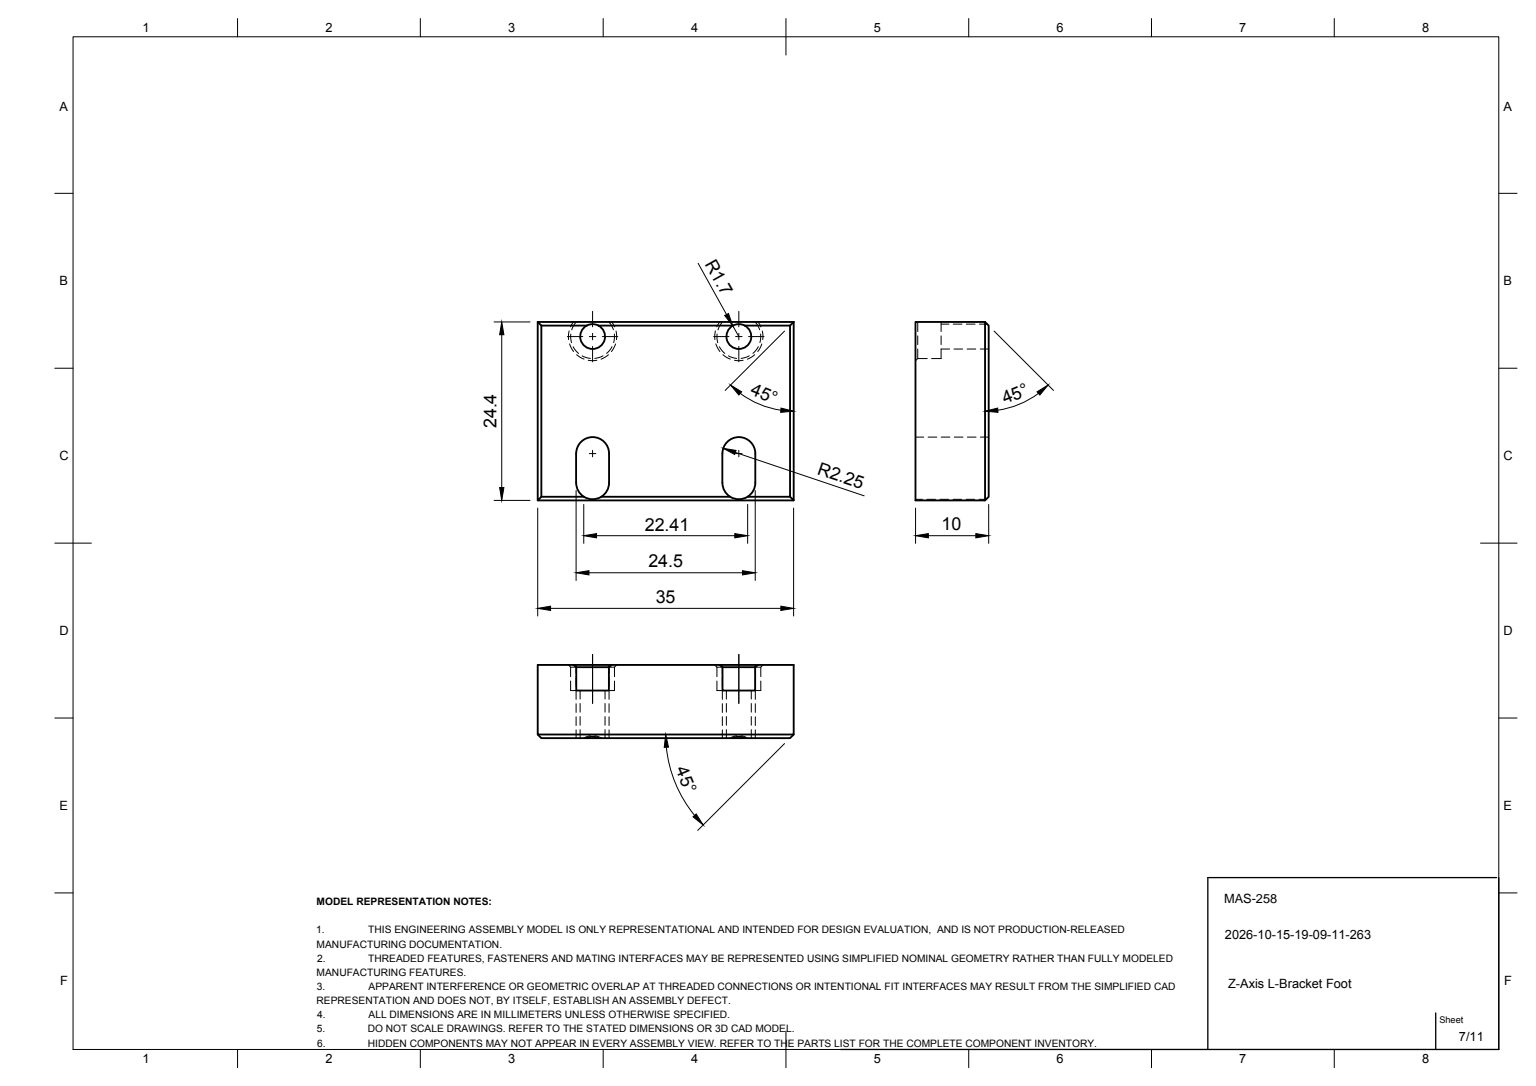
ISO-10303-21;
HEADER;
/* Generated by software containing ST-Developer
 * from STEP Tools, Inc. (www.steptools.com) 
 */

FILE_DESCRIPTION(
/* description */ (''),
/* implementation_level */ '2;1');

FILE_NAME(
/* name */ 'Z-Axis L-Bracket Foot.step',
/* time_stamp */ '2026-10-15T12:29:06-07:00',
/* author */ (''),
/* organization */ (''),
/* preprocessor_version */ 'ST-DEVELOPER v20.2',
/* originating_system */ 'Autodesk Translation Framework v15.15.0.0',
/* authorisation */ '');

FILE_SCHEMA (('AUTOMOTIVE_DESIGN { 1 0 10303 214 3 1 1 }'));
ENDSEC;

DATA;
#10=MECHANICAL_DESIGN_GEOMETRIC_PRESENTATION_REPRESENTATION('',(#1746),#135282);
#100=(
BOUNDED_CURVE()
B_SPLINE_CURVE(2,(#76990,#76991,#76992),.UNSPECIFIED.,.F.,.F.)
B_SPLINE_CURVE_WITH_KNOTS((3,3),(0.557415897727321,0.585832740635072),
 .UNSPECIFIED.)
CURVE()
GEOMETRIC_REPRESENTATION_ITEM()
RATIONAL_B_SPLINE_CURVE((1.06,1.03152938818342,1.))
REPRESENTATION_ITEM('')
);
#101=(
BOUNDED_CURVE()
B_SPLINE_CURVE(2,(#76996,#76997,#76998),.UNSPECIFIED.,.F.,.F.)
B_SPLINE_CURVE_WITH_KNOTS((3,3),(0.,0.0284168429077509),.UNSPECIFIED.)
CURVE()
GEOMETRIC_REPRESENTATION_ITEM()
RATIONAL_B_SPLINE_CURVE((1.,1.03152938818342,1.06))
REPRESENTATION_ITEM('')
);
#102=(
BOUNDED_CURVE()
B_SPLINE_CURVE(2,(#77032,#77033,#77034),.UNSPECIFIED.,.F.,.F.)
B_SPLINE_CURVE_WITH_KNOTS((3,3),(0.557415897727321,0.585832740635072),
 .UNSPECIFIED.)
CURVE()
GEOMETRIC_REPRESENTATION_ITEM()
RATIONAL_B_SPLINE_CURVE((1.06,1.03152938818342,1.))
REPRESENTATION_ITEM('')
);
#103=(
BOUNDED_CURVE()
B_SPLINE_CURVE(2,(#77036,#77037,#77038),.UNSPECIFIED.,.F.,.F.)
B_SPLINE_CURVE_WITH_KNOTS((3,3),(0.,0.028416842907751),.UNSPECIFIED.)
CURVE()
GEOMETRIC_REPRESENTATION_ITEM()
RATIONAL_B_SPLINE_CURVE((1.,1.03152938818342,1.06))
REPRESENTATION_ITEM('')
);
#300=ELLIPSE('',#33382,2.40416305603426,1.7);
#301=ELLIPSE('',#33386,2.40416305603426,1.7);
#302=ELLIPSE('',#33391,3.18198051533946,2.25);
#303=ELLIPSE('',#33399,3.18198051533947,2.25);
#1720=SHAPE_REPRESENTATION_RELATIONSHIP('SRR','None',#135344,#1733);
#1733=ADVANCED_BREP_SHAPE_REPRESENTATION('',(#1759),#135276);
#1746=STYLED_ITEM('',(#135418),#1759);
#1759=MANIFOLD_SOLID_BREP('Body1',#32082);
#1848=CYLINDRICAL_SURFACE('',#33372,3.);
#1849=CYLINDRICAL_SURFACE('',#33376,3.);
#1850=CYLINDRICAL_SURFACE('',#33380,1.7);
#1851=CYLINDRICAL_SURFACE('',#33384,1.7);
#1852=CYLINDRICAL_SURFACE('',#33390,2.25);
#1853=CYLINDRICAL_SURFACE('',#33395,2.25);
#1854=CYLINDRICAL_SURFACE('',#33398,2.25);
#1855=CYLINDRICAL_SURFACE('',#33403,2.25);
#2210=FACE_BOUND('',#6520,.T.);
#2211=FACE_BOUND('',#6521,.T.);
#2212=FACE_BOUND('',#6526,.T.);
#2213=FACE_BOUND('',#6529,.T.);
#3026=PLANE('',#33363);
#3027=PLANE('',#33371);
#3028=PLANE('',#33374);
#3029=PLANE('',#33378);
#3030=PLANE('',#33388);
#3031=PLANE('',#33389);
#3032=PLANE('',#33394);
#3033=PLANE('',#33397);
#3034=PLANE('',#33402);
#3035=PLANE('',#33405);
#3036=PLANE('',#33406);
#3037=PLANE('',#33407);
#3038=PLANE('',#33408);
#3039=PLANE('',#33409);
#3040=PLANE('',#33410);
#3041=PLANE('',#33411);
#4570=FACE_OUTER_BOUND('',#6518,.T.);
#4571=FACE_OUTER_BOUND('',#6519,.T.);
#4572=FACE_OUTER_BOUND('',#6522,.T.);
#4573=FACE_OUTER_BOUND('',#6523,.T.);
#4574=FACE_OUTER_BOUND('',#6524,.T.);
#4575=FACE_OUTER_BOUND('',#6525,.T.);
#4576=FACE_OUTER_BOUND('',#6527,.T.);
#4577=FACE_OUTER_BOUND('',#6528,.T.);
#4578=FACE_OUTER_BOUND('',#6530,.T.);
#4579=FACE_OUTER_BOUND('',#6531,.T.);
#4580=FACE_OUTER_BOUND('',#6532,.T.);
#4581=FACE_OUTER_BOUND('',#6533,.T.);
#4582=FACE_OUTER_BOUND('',#6534,.T.);
#4583=FACE_OUTER_BOUND('',#6535,.T.);
#4584=FACE_OUTER_BOUND('',#6536,.T.);
#4585=FACE_OUTER_BOUND('',#6537,.T.);
#4586=FACE_OUTER_BOUND('',#6538,.T.);
#4587=FACE_OUTER_BOUND('',#6539,.T.);
#4588=FACE_OUTER_BOUND('',#6540,.T.);
#4589=FACE_OUTER_BOUND('',#6541,.T.);
#4590=FACE_OUTER_BOUND('',#6542,.T.);
#4591=FACE_OUTER_BOUND('',#6543,.T.);
#4592=FACE_OUTER_BOUND('',#6544,.T.);
#4593=FACE_OUTER_BOUND('',#6545,.T.);
#4594=FACE_OUTER_BOUND('',#6546,.T.);
#4595=FACE_OUTER_BOUND('',#6547,.T.);
#6518=EDGE_LOOP('',(#27186,#27187,#27188,#27189));
#6519=EDGE_LOOP('',(#27190,#27191,#27192,#27193,#27194,#27195,#27196,#27197));
#6520=EDGE_LOOP('',(#27198,#27199,#27200,#27201));
#6521=EDGE_LOOP('',(#27202,#27203,#27204,#27205));
#6522=EDGE_LOOP('',(#27206,#27207,#27208,#27209));
#6523=EDGE_LOOP('',(#27210,#27211,#27212,#27213,#27214,#27215,#27216,#27217,
#27218,#27219,#27220,#27221,#27222,#27223,#27224,#27225));
#6524=EDGE_LOOP('',(#27226,#27227,#27228,#27229));
#6525=EDGE_LOOP('',(#27230,#27231));
#6526=EDGE_LOOP('',(#27232));
#6527=EDGE_LOOP('',(#27233,#27234,#27235,#27236));
#6528=EDGE_LOOP('',(#27237,#27238));
#6529=EDGE_LOOP('',(#27239));
#6530=EDGE_LOOP('',(#27240,#27241,#27242,#27243,#27244,#27245));
#6531=EDGE_LOOP('',(#27246,#27247,#27248,#27249,#27250,#27251));
#6532=EDGE_LOOP('',(#27252,#27253,#27254,#27255,#27256,#27257,#27258,#27259));
#6533=EDGE_LOOP('',(#27260,#27261,#27262,#27263));
#6534=EDGE_LOOP('',(#27264,#27265,#27266,#27267,#27268,#27269));
#6535=EDGE_LOOP('',(#27270,#27271,#27272,#27273));
#6536=EDGE_LOOP('',(#27274,#27275,#27276,#27277));
#6537=EDGE_LOOP('',(#27278,#27279,#27280,#27281));
#6538=EDGE_LOOP('',(#27282,#27283,#27284,#27285,#27286,#27287));
#6539=EDGE_LOOP('',(#27288,#27289,#27290,#27291));
#6540=EDGE_LOOP('',(#27292,#27293,#27294,#27295));
#6541=EDGE_LOOP('',(#27296,#27297,#27298,#27299,#27300,#27301,#27302,#27303,
#27304,#27305,#27306,#27307,#27308,#27309,#27310,#27311,#27312,#27313,#27314,
#27315,#27316,#27317));
#6542=EDGE_LOOP('',(#27318,#27319,#27320,#27321));
#6543=EDGE_LOOP('',(#27322,#27323,#27324,#27325));
#6544=EDGE_LOOP('',(#27326,#27327,#27328,#27329,#27330,#27331,#27332,#27333));
#6545=EDGE_LOOP('',(#27334,#27335,#27336,#27337));
#6546=EDGE_LOOP('',(#27338,#27339,#27340,#27341));
#6547=EDGE_LOOP('',(#27342,#27343,#27344,#27345));
#9216=LINE('',#77002,#12053);
#9217=LINE('',#77006,#12054);
#9218=LINE('',#77008,#12055);
#9219=LINE('',#77010,#12056);
#9220=LINE('',#77012,#12057);
#9221=LINE('',#77013,#12058);
#9222=LINE('',#77016,#12059);
#9223=LINE('',#77020,#12060);
#9224=LINE('',#77024,#12061);
#9225=LINE('',#77028,#12062);
#9226=LINE('',#77042,#12063);
#9227=LINE('',#77044,#12064);
#9228=LINE('',#77045,#12065);
#9229=LINE('',#77047,#12066);
#9230=LINE('',#77049,#12067);
#9231=LINE('',#77050,#12068);
#9232=LINE('',#77052,#12069);
#9233=LINE('',#77054,#12070);
#9234=LINE('',#77055,#12071);
#9235=LINE('',#77068,#12072);
#9236=LINE('',#77076,#12073);
#9237=LINE('',#77084,#12074);
#9238=LINE('',#77085,#12075);
#9239=LINE('',#77087,#12076);
#9240=LINE('',#77088,#12077);
#9241=LINE('',#77089,#12078);
#9242=LINE('',#77093,#12079);
#9243=LINE('',#77094,#12080);
#9244=LINE('',#77095,#12081);
#9245=LINE('',#77102,#12082);
#9246=LINE('',#77106,#12083);
#9247=LINE('',#77107,#12084);
#9248=LINE('',#77113,#12085);
#9249=LINE('',#77114,#12086);
#9250=LINE('',#77115,#12087);
#9251=LINE('',#77122,#12088);
#9252=LINE('',#77126,#12089);
#9253=LINE('',#77127,#12090);
#9254=LINE('',#77132,#12091);
#9255=LINE('',#77133,#12092);
#9256=LINE('',#77134,#12093);
#9257=LINE('',#77136,#12094);
#9258=LINE('',#77137,#12095);
#9259=LINE('',#77140,#12096);
#9260=LINE('',#77141,#12097);
#9261=LINE('',#77144,#12098);
#9262=LINE('',#77145,#12099);
#9263=LINE('',#77147,#12100);
#9264=LINE('',#77149,#12101);
#9265=LINE('',#77150,#12102);
#12053=VECTOR('',#38634,10.);
#12054=VECTOR('',#38637,10.);
#12055=VECTOR('',#38638,10.);
#12056=VECTOR('',#38639,10.);
#12057=VECTOR('',#38640,10.);
#12058=VECTOR('',#38641,10.);
#12059=VECTOR('',#38642,10.);
#12060=VECTOR('',#38645,10.);
#12061=VECTOR('',#38648,10.);
#12062=VECTOR('',#38651,10.);
#12063=VECTOR('',#38660,10.);
#12064=VECTOR('',#38661,10.);
#12065=VECTOR('',#38662,10.);
#12066=VECTOR('',#38663,10.);
#12067=VECTOR('',#38664,10.);
#12068=VECTOR('',#38665,10.);
#12069=VECTOR('',#38666,10.);
#12070=VECTOR('',#38667,10.);
#12071=VECTOR('',#38668,10.);
#12072=VECTOR('',#38687,1.7);
#12073=VECTOR('',#38696,1.7);
#12074=VECTOR('',#38705,10.);
#12075=VECTOR('',#38706,10.);
#12076=VECTOR('',#38707,10.);
#12077=VECTOR('',#38708,10.);
#12078=VECTOR('',#38709,10.);
#12079=VECTOR('',#38712,10.);
#12080=VECTOR('',#38713,10.);
#12081=VECTOR('',#38714,10.);
#12082=VECTOR('',#38721,10.);
#12083=VECTOR('',#38726,10.);
#12084=VECTOR('',#38727,10.);
#12085=VECTOR('',#38734,10.);
#12086=VECTOR('',#38735,10.);
#12087=VECTOR('',#38736,10.);
#12088=VECTOR('',#38743,10.);
#12089=VECTOR('',#38748,10.);
#12090=VECTOR('',#38749,10.);
#12091=VECTOR('',#38756,10.);
#12092=VECTOR('',#38757,10.);
#12093=VECTOR('',#38758,10.);
#12094=VECTOR('',#38759,10.);
#12095=VECTOR('',#38760,10.);
#12096=VECTOR('',#38763,10.);
#12097=VECTOR('',#38764,10.);
#12098=VECTOR('',#38767,10.);
#12099=VECTOR('',#38768,10.);
#12100=VECTOR('',#38771,10.);
#12101=VECTOR('',#38774,10.);
#12102=VECTOR('',#38775,10.);
#12932=CIRCLE('',#33361,3.3);
#12933=CIRCLE('',#33362,3.);
#12934=CIRCLE('',#33364,3.3);
#12935=CIRCLE('',#33365,2.25);
#12936=CIRCLE('',#33366,2.25);
#12937=CIRCLE('',#33367,2.25);
#12938=CIRCLE('',#33368,2.25);
#12939=CIRCLE('',#33370,3.);
#12940=CIRCLE('',#33373,3.);
#12941=CIRCLE('',#33375,1.7);
#12942=CIRCLE('',#33377,3.);
#12943=CIRCLE('',#33379,1.7);
#12944=CIRCLE('',#33381,1.7);
#12945=CIRCLE('',#33383,1.7);
#12946=CIRCLE('',#33385,1.7);
#12947=CIRCLE('',#33387,1.7);
#12948=CIRCLE('',#33392,2.25);
#12949=CIRCLE('',#33393,2.25);
#12950=CIRCLE('',#33396,2.25);
#12951=CIRCLE('',#33400,2.25);
#12952=CIRCLE('',#33401,2.25);
#12953=CIRCLE('',#33404,2.25);
#15317=VERTEX_POINT('',#76988);
#15318=VERTEX_POINT('',#76989);
#15319=VERTEX_POINT('',#76993);
#15320=VERTEX_POINT('',#76995);
#15321=VERTEX_POINT('',#77001);
#15322=VERTEX_POINT('',#77003);
#15323=VERTEX_POINT('',#77005);
#15324=VERTEX_POINT('',#77007);
#15325=VERTEX_POINT('',#77009);
#15326=VERTEX_POINT('',#77011);
#15327=VERTEX_POINT('',#77014);
#15328=VERTEX_POINT('',#77015);
#15329=VERTEX_POINT('',#77017);
#15330=VERTEX_POINT('',#77019);
#15331=VERTEX_POINT('',#77022);
#15332=VERTEX_POINT('',#77023);
#15333=VERTEX_POINT('',#77025);
#15334=VERTEX_POINT('',#77027);
#15335=VERTEX_POINT('',#77031);
#15336=VERTEX_POINT('',#77035);
#15337=VERTEX_POINT('',#77041);
#15338=VERTEX_POINT('',#77043);
#15339=VERTEX_POINT('',#77046);
#15340=VERTEX_POINT('',#77048);
#15341=VERTEX_POINT('',#77051);
#15342=VERTEX_POINT('',#77053);
#15343=VERTEX_POINT('',#77059);
#15344=VERTEX_POINT('',#77064);
#15345=VERTEX_POINT('',#77067);
#15346=VERTEX_POINT('',#77069);
#15347=VERTEX_POINT('',#77071);
#15348=VERTEX_POINT('',#77075);
#15349=VERTEX_POINT('',#77077);
#15350=VERTEX_POINT('',#77079);
#15351=VERTEX_POINT('',#77083);
#15352=VERTEX_POINT('',#77086);
#15353=VERTEX_POINT('',#77091);
#15354=VERTEX_POINT('',#77092);
#15355=VERTEX_POINT('',#77097);
#15356=VERTEX_POINT('',#77098);
#15357=VERTEX_POINT('',#77100);
#15358=VERTEX_POINT('',#77105);
#15359=VERTEX_POINT('',#77111);
#15360=VERTEX_POINT('',#77112);
#15361=VERTEX_POINT('',#77117);
#15362=VERTEX_POINT('',#77118);
#15363=VERTEX_POINT('',#77120);
#15364=VERTEX_POINT('',#77125);
#15365=VERTEX_POINT('',#77131);
#15366=VERTEX_POINT('',#77135);
#15367=VERTEX_POINT('',#77139);
#15368=VERTEX_POINT('',#77143);
#19444=EDGE_CURVE('',#15317,#15318,#100,.T.);
#19445=EDGE_CURVE('',#15318,#15319,#12932,.T.);
#19446=EDGE_CURVE('',#15319,#15320,#101,.T.);
#19447=EDGE_CURVE('',#15320,#15317,#12933,.T.);
#19448=EDGE_CURVE('',#15318,#15321,#9216,.T.);
#19449=EDGE_CURVE('',#15322,#15321,#12934,.T.);
#19450=EDGE_CURVE('',#15322,#15323,#9217,.T.);
#19451=EDGE_CURVE('',#15323,#15324,#9218,.T.);
#19452=EDGE_CURVE('',#15324,#15325,#9219,.T.);
#19453=EDGE_CURVE('',#15325,#15326,#9220,.T.);
#19454=EDGE_CURVE('',#15326,#15319,#9221,.T.);
#19455=EDGE_CURVE('',#15327,#15328,#9222,.T.);
#19456=EDGE_CURVE('',#15328,#15329,#12935,.T.);
#19457=EDGE_CURVE('',#15329,#15330,#9223,.T.);
#19458=EDGE_CURVE('',#15330,#15327,#12936,.T.);
#19459=EDGE_CURVE('',#15331,#15332,#9224,.T.);
#19460=EDGE_CURVE('',#15332,#15333,#12937,.T.);
#19461=EDGE_CURVE('',#15333,#15334,#9225,.T.);
#19462=EDGE_CURVE('',#15334,#15331,#12938,.T.);
#19463=EDGE_CURVE('',#15335,#15322,#102,.T.);
#19464=EDGE_CURVE('',#15321,#15336,#103,.T.);
#19465=EDGE_CURVE('',#15336,#15335,#12939,.T.);
#19466=EDGE_CURVE('',#15326,#15337,#9226,.T.);
#19467=EDGE_CURVE('',#15338,#15337,#9227,.T.);
#19468=EDGE_CURVE('',#15323,#15338,#9228,.T.);
#19469=EDGE_CURVE('',#15335,#15339,#9229,.T.);
#19470=EDGE_CURVE('',#15339,#15340,#9230,.T.);
#19471=EDGE_CURVE('',#15340,#15336,#9231,.T.);
#19472=EDGE_CURVE('',#15317,#15341,#9232,.T.);
#19473=EDGE_CURVE('',#15341,#15342,#9233,.T.);
#19474=EDGE_CURVE('',#15342,#15320,#9234,.T.);
#19475=EDGE_CURVE('',#15340,#15339,#12940,.T.);
#19476=EDGE_CURVE('',#15343,#15343,#12941,.T.);
#19477=EDGE_CURVE('',#15342,#15341,#12942,.T.);
#19478=EDGE_CURVE('',#15344,#15344,#12943,.T.);
#19479=EDGE_CURVE('',#15343,#15345,#9235,.T.);
#19480=EDGE_CURVE('',#15346,#15345,#12944,.T.);
#19481=EDGE_CURVE('',#15347,#15346,#300,.T.);
#19482=EDGE_CURVE('',#15345,#15347,#12945,.T.);
#19483=EDGE_CURVE('',#15344,#15348,#9236,.T.);
#19484=EDGE_CURVE('',#15349,#15348,#12946,.T.);
#19485=EDGE_CURVE('',#15350,#15349,#301,.T.);
#19486=EDGE_CURVE('',#15348,#15350,#12947,.T.);
#19487=EDGE_CURVE('',#15346,#15351,#9237,.T.);
#19488=EDGE_CURVE('',#15351,#15338,#9238,.T.);
#19489=EDGE_CURVE('',#15352,#15337,#9239,.T.);
#19490=EDGE_CURVE('',#15352,#15350,#9240,.T.);
#19491=EDGE_CURVE('',#15349,#15347,#9241,.T.);
#19492=EDGE_CURVE('',#15353,#15354,#9242,.T.);
#19493=EDGE_CURVE('',#15353,#15332,#9243,.T.);
#19494=EDGE_CURVE('',#15354,#15331,#9244,.T.);
#19495=EDGE_CURVE('',#15355,#15356,#302,.T.);
#19496=EDGE_CURVE('',#15357,#15355,#12948,.T.);
#19497=EDGE_CURVE('',#15357,#15333,#9245,.T.);
#19498=EDGE_CURVE('',#15356,#15353,#12949,.T.);
#19499=EDGE_CURVE('',#15358,#15357,#9246,.T.);
#19500=EDGE_CURVE('',#15358,#15334,#9247,.T.);
#19501=EDGE_CURVE('',#15354,#15358,#12950,.T.);
#19502=EDGE_CURVE('',#15359,#15360,#9248,.T.);
#19503=EDGE_CURVE('',#15359,#15328,#9249,.T.);
#19504=EDGE_CURVE('',#15360,#15327,#9250,.T.);
#19505=EDGE_CURVE('',#15361,#15362,#303,.T.);
#19506=EDGE_CURVE('',#15363,#15361,#12951,.T.);
#19507=EDGE_CURVE('',#15363,#15329,#9251,.T.);
#19508=EDGE_CURVE('',#15362,#15359,#12952,.T.);
#19509=EDGE_CURVE('',#15364,#15363,#9252,.T.);
#19510=EDGE_CURVE('',#15364,#15330,#9253,.T.);
#19511=EDGE_CURVE('',#15360,#15364,#12953,.T.);
#19512=EDGE_CURVE('',#15365,#15352,#9254,.T.);
#19513=EDGE_CURVE('',#15362,#15365,#9255,.T.);
#19514=EDGE_CURVE('',#15356,#15361,#9256,.T.);
#19515=EDGE_CURVE('',#15366,#15355,#9257,.T.);
#19516=EDGE_CURVE('',#15351,#15366,#9258,.T.);
#19517=EDGE_CURVE('',#15337,#15367,#9259,.T.);
#19518=EDGE_CURVE('',#15365,#15367,#9260,.T.);
#19519=EDGE_CURVE('',#15366,#15368,#9261,.T.);
#19520=EDGE_CURVE('',#15368,#15338,#9262,.T.);
#19521=EDGE_CURVE('',#15367,#15368,#9263,.T.);
#19522=EDGE_CURVE('',#15325,#15367,#9264,.T.);
#19523=EDGE_CURVE('',#15324,#15368,#9265,.T.);
#27186=ORIENTED_EDGE('',*,*,#19444,.T.);
#27187=ORIENTED_EDGE('',*,*,#19445,.T.);
#27188=ORIENTED_EDGE('',*,*,#19446,.T.);
#27189=ORIENTED_EDGE('',*,*,#19447,.T.);
#27190=ORIENTED_EDGE('',*,*,#19445,.F.);
#27191=ORIENTED_EDGE('',*,*,#19448,.T.);
#27192=ORIENTED_EDGE('',*,*,#19449,.F.);
#27193=ORIENTED_EDGE('',*,*,#19450,.T.);
#27194=ORIENTED_EDGE('',*,*,#19451,.T.);
#27195=ORIENTED_EDGE('',*,*,#19452,.T.);
#27196=ORIENTED_EDGE('',*,*,#19453,.T.);
#27197=ORIENTED_EDGE('',*,*,#19454,.T.);
#27198=ORIENTED_EDGE('',*,*,#19455,.T.);
#27199=ORIENTED_EDGE('',*,*,#19456,.T.);
#27200=ORIENTED_EDGE('',*,*,#19457,.T.);
#27201=ORIENTED_EDGE('',*,*,#19458,.T.);
#27202=ORIENTED_EDGE('',*,*,#19459,.T.);
#27203=ORIENTED_EDGE('',*,*,#19460,.T.);
#27204=ORIENTED_EDGE('',*,*,#19461,.T.);
#27205=ORIENTED_EDGE('',*,*,#19462,.T.);
#27206=ORIENTED_EDGE('',*,*,#19463,.T.);
#27207=ORIENTED_EDGE('',*,*,#19449,.T.);
#27208=ORIENTED_EDGE('',*,*,#19464,.T.);
#27209=ORIENTED_EDGE('',*,*,#19465,.T.);
#27210=ORIENTED_EDGE('',*,*,#19446,.F.);
#27211=ORIENTED_EDGE('',*,*,#19454,.F.);
#27212=ORIENTED_EDGE('',*,*,#19466,.T.);
#27213=ORIENTED_EDGE('',*,*,#19467,.F.);
#27214=ORIENTED_EDGE('',*,*,#19468,.F.);
#27215=ORIENTED_EDGE('',*,*,#19450,.F.);
#27216=ORIENTED_EDGE('',*,*,#19463,.F.);
#27217=ORIENTED_EDGE('',*,*,#19469,.T.);
#27218=ORIENTED_EDGE('',*,*,#19470,.T.);
#27219=ORIENTED_EDGE('',*,*,#19471,.T.);
#27220=ORIENTED_EDGE('',*,*,#19464,.F.);
#27221=ORIENTED_EDGE('',*,*,#19448,.F.);
#27222=ORIENTED_EDGE('',*,*,#19444,.F.);
#27223=ORIENTED_EDGE('',*,*,#19472,.T.);
#27224=ORIENTED_EDGE('',*,*,#19473,.T.);
#27225=ORIENTED_EDGE('',*,*,#19474,.T.);
#27226=ORIENTED_EDGE('',*,*,#19465,.F.);
#27227=ORIENTED_EDGE('',*,*,#19471,.F.);
#27228=ORIENTED_EDGE('',*,*,#19475,.T.);
#27229=ORIENTED_EDGE('',*,*,#19469,.F.);
#27230=ORIENTED_EDGE('',*,*,#19470,.F.);
#27231=ORIENTED_EDGE('',*,*,#19475,.F.);
#27232=ORIENTED_EDGE('',*,*,#19476,.F.);
#27233=ORIENTED_EDGE('',*,*,#19447,.F.);
#27234=ORIENTED_EDGE('',*,*,#19474,.F.);
#27235=ORIENTED_EDGE('',*,*,#19477,.T.);
#27236=ORIENTED_EDGE('',*,*,#19472,.F.);
#27237=ORIENTED_EDGE('',*,*,#19473,.F.);
#27238=ORIENTED_EDGE('',*,*,#19477,.F.);
#27239=ORIENTED_EDGE('',*,*,#19478,.F.);
#27240=ORIENTED_EDGE('',*,*,#19476,.T.);
#27241=ORIENTED_EDGE('',*,*,#19479,.T.);
#27242=ORIENTED_EDGE('',*,*,#19480,.F.);
#27243=ORIENTED_EDGE('',*,*,#19481,.F.);
#27244=ORIENTED_EDGE('',*,*,#19482,.F.);
#27245=ORIENTED_EDGE('',*,*,#19479,.F.);
#27246=ORIENTED_EDGE('',*,*,#19478,.T.);
#27247=ORIENTED_EDGE('',*,*,#19483,.T.);
#27248=ORIENTED_EDGE('',*,*,#19484,.F.);
#27249=ORIENTED_EDGE('',*,*,#19485,.F.);
#27250=ORIENTED_EDGE('',*,*,#19486,.F.);
#27251=ORIENTED_EDGE('',*,*,#19483,.F.);
#27252=ORIENTED_EDGE('',*,*,#19481,.T.);
#27253=ORIENTED_EDGE('',*,*,#19487,.T.);
#27254=ORIENTED_EDGE('',*,*,#19488,.T.);
#27255=ORIENTED_EDGE('',*,*,#19467,.T.);
#27256=ORIENTED_EDGE('',*,*,#19489,.F.);
#27257=ORIENTED_EDGE('',*,*,#19490,.T.);
#27258=ORIENTED_EDGE('',*,*,#19485,.T.);
#27259=ORIENTED_EDGE('',*,*,#19491,.T.);
#27260=ORIENTED_EDGE('',*,*,#19492,.F.);
#27261=ORIENTED_EDGE('',*,*,#19493,.T.);
#27262=ORIENTED_EDGE('',*,*,#19459,.F.);
#27263=ORIENTED_EDGE('',*,*,#19494,.F.);
#27264=ORIENTED_EDGE('',*,*,#19495,.F.);
#27265=ORIENTED_EDGE('',*,*,#19496,.F.);
#27266=ORIENTED_EDGE('',*,*,#19497,.T.);
#27267=ORIENTED_EDGE('',*,*,#19460,.F.);
#27268=ORIENTED_EDGE('',*,*,#19493,.F.);
#27269=ORIENTED_EDGE('',*,*,#19498,.F.);
#27270=ORIENTED_EDGE('',*,*,#19499,.F.);
#27271=ORIENTED_EDGE('',*,*,#19500,.T.);
#27272=ORIENTED_EDGE('',*,*,#19461,.F.);
#27273=ORIENTED_EDGE('',*,*,#19497,.F.);
#27274=ORIENTED_EDGE('',*,*,#19501,.F.);
#27275=ORIENTED_EDGE('',*,*,#19494,.T.);
#27276=ORIENTED_EDGE('',*,*,#19462,.F.);
#27277=ORIENTED_EDGE('',*,*,#19500,.F.);
#27278=ORIENTED_EDGE('',*,*,#19502,.F.);
#27279=ORIENTED_EDGE('',*,*,#19503,.T.);
#27280=ORIENTED_EDGE('',*,*,#19455,.F.);
#27281=ORIENTED_EDGE('',*,*,#19504,.F.);
#27282=ORIENTED_EDGE('',*,*,#19505,.F.);
#27283=ORIENTED_EDGE('',*,*,#19506,.F.);
#27284=ORIENTED_EDGE('',*,*,#19507,.T.);
#27285=ORIENTED_EDGE('',*,*,#19456,.F.);
#27286=ORIENTED_EDGE('',*,*,#19503,.F.);
#27287=ORIENTED_EDGE('',*,*,#19508,.F.);
#27288=ORIENTED_EDGE('',*,*,#19509,.F.);
#27289=ORIENTED_EDGE('',*,*,#19510,.T.);
#27290=ORIENTED_EDGE('',*,*,#19457,.F.);
#27291=ORIENTED_EDGE('',*,*,#19507,.F.);
#27292=ORIENTED_EDGE('',*,*,#19511,.F.);
#27293=ORIENTED_EDGE('',*,*,#19504,.T.);
#27294=ORIENTED_EDGE('',*,*,#19458,.F.);
#27295=ORIENTED_EDGE('',*,*,#19510,.F.);
#27296=ORIENTED_EDGE('',*,*,#19480,.T.);
#27297=ORIENTED_EDGE('',*,*,#19482,.T.);
#27298=ORIENTED_EDGE('',*,*,#19491,.F.);
#27299=ORIENTED_EDGE('',*,*,#19484,.T.);
#27300=ORIENTED_EDGE('',*,*,#19486,.T.);
#27301=ORIENTED_EDGE('',*,*,#19490,.F.);
#27302=ORIENTED_EDGE('',*,*,#19512,.F.);
#27303=ORIENTED_EDGE('',*,*,#19513,.F.);
#27304=ORIENTED_EDGE('',*,*,#19508,.T.);
#27305=ORIENTED_EDGE('',*,*,#19502,.T.);
#27306=ORIENTED_EDGE('',*,*,#19511,.T.);
#27307=ORIENTED_EDGE('',*,*,#19509,.T.);
#27308=ORIENTED_EDGE('',*,*,#19506,.T.);
#27309=ORIENTED_EDGE('',*,*,#19514,.F.);
#27310=ORIENTED_EDGE('',*,*,#19498,.T.);
#27311=ORIENTED_EDGE('',*,*,#19492,.T.);
#27312=ORIENTED_EDGE('',*,*,#19501,.T.);
#27313=ORIENTED_EDGE('',*,*,#19499,.T.);
#27314=ORIENTED_EDGE('',*,*,#19496,.T.);
#27315=ORIENTED_EDGE('',*,*,#19515,.F.);
#27316=ORIENTED_EDGE('',*,*,#19516,.F.);
#27317=ORIENTED_EDGE('',*,*,#19487,.F.);
#27318=ORIENTED_EDGE('',*,*,#19512,.T.);
#27319=ORIENTED_EDGE('',*,*,#19489,.T.);
#27320=ORIENTED_EDGE('',*,*,#19517,.T.);
#27321=ORIENTED_EDGE('',*,*,#19518,.F.);
#27322=ORIENTED_EDGE('',*,*,#19516,.T.);
#27323=ORIENTED_EDGE('',*,*,#19519,.T.);
#27324=ORIENTED_EDGE('',*,*,#19520,.T.);
#27325=ORIENTED_EDGE('',*,*,#19488,.F.);
#27326=ORIENTED_EDGE('',*,*,#19495,.T.);
#27327=ORIENTED_EDGE('',*,*,#19514,.T.);
#27328=ORIENTED_EDGE('',*,*,#19505,.T.);
#27329=ORIENTED_EDGE('',*,*,#19513,.T.);
#27330=ORIENTED_EDGE('',*,*,#19518,.T.);
#27331=ORIENTED_EDGE('',*,*,#19521,.T.);
#27332=ORIENTED_EDGE('',*,*,#19519,.F.);
#27333=ORIENTED_EDGE('',*,*,#19515,.T.);
#27334=ORIENTED_EDGE('',*,*,#19521,.F.);
#27335=ORIENTED_EDGE('',*,*,#19522,.F.);
#27336=ORIENTED_EDGE('',*,*,#19452,.F.);
#27337=ORIENTED_EDGE('',*,*,#19523,.T.);
#27338=ORIENTED_EDGE('',*,*,#19517,.F.);
#27339=ORIENTED_EDGE('',*,*,#19466,.F.);
#27340=ORIENTED_EDGE('',*,*,#19453,.F.);
#27341=ORIENTED_EDGE('',*,*,#19522,.T.);
#27342=ORIENTED_EDGE('',*,*,#19520,.F.);
#27343=ORIENTED_EDGE('',*,*,#19523,.F.);
#27344=ORIENTED_EDGE('',*,*,#19451,.F.);
#27345=ORIENTED_EDGE('',*,*,#19468,.T.);
#30292=CONICAL_SURFACE('',#33360,3.15,0.785398163397449);
#30293=CONICAL_SURFACE('',#33369,3.15,0.785398163397449);
#31545=ADVANCED_FACE('',(#4570),#30292,.F.);
#31546=ADVANCED_FACE('',(#4571,#2210,#2211),#3026,.F.);
#31547=ADVANCED_FACE('',(#4572),#30293,.F.);
#31548=ADVANCED_FACE('',(#4573),#3027,.T.);
#31549=ADVANCED_FACE('',(#4574),#1848,.F.);
#31550=ADVANCED_FACE('',(#4575,#2212),#3028,.F.);
#31551=ADVANCED_FACE('',(#4576),#1849,.F.);
#31552=ADVANCED_FACE('',(#4577,#2213),#3029,.F.);
#31553=ADVANCED_FACE('',(#4578),#1850,.F.);
#31554=ADVANCED_FACE('',(#4579),#1851,.F.);
#31555=ADVANCED_FACE('',(#4580),#3030,.T.);
#31556=ADVANCED_FACE('',(#4581),#3031,.F.);
#31557=ADVANCED_FACE('',(#4582),#1852,.F.);
#31558=ADVANCED_FACE('',(#4583),#3032,.F.);
#31559=ADVANCED_FACE('',(#4584),#1853,.F.);
#31560=ADVANCED_FACE('',(#4585),#3033,.F.);
#31561=ADVANCED_FACE('',(#4586),#1854,.F.);
#31562=ADVANCED_FACE('',(#4587),#3034,.F.);
#31563=ADVANCED_FACE('',(#4588),#1855,.F.);
#31564=ADVANCED_FACE('',(#4589),#3035,.T.);
#31565=ADVANCED_FACE('',(#4590),#3036,.T.);
#31566=ADVANCED_FACE('',(#4591),#3037,.T.);
#31567=ADVANCED_FACE('',(#4592),#3038,.T.);
#31568=ADVANCED_FACE('',(#4593),#3039,.T.);
#31569=ADVANCED_FACE('',(#4594),#3040,.T.);
#31570=ADVANCED_FACE('',(#4595),#3041,.T.);
#32082=CLOSED_SHELL('',(#31545,#31546,#31547,#31548,#31549,#31550,#31551,
#31552,#31553,#31554,#31555,#31556,#31557,#31558,#31559,#31560,#31561,#31562,
#31563,#31564,#31565,#31566,#31567,#31568,#31569,#31570));
#33359=AXIS2_PLACEMENT_3D('',#76986,#38624,#38625);
#33360=AXIS2_PLACEMENT_3D('',#76987,#38626,#38627);
#33361=AXIS2_PLACEMENT_3D('',#76994,#38628,#38629);
#33362=AXIS2_PLACEMENT_3D('',#76999,#38630,#38631);
#33363=AXIS2_PLACEMENT_3D('',#77000,#38632,#38633);
#33364=AXIS2_PLACEMENT_3D('',#77004,#38635,#38636);
#33365=AXIS2_PLACEMENT_3D('',#77018,#38643,#38644);
#33366=AXIS2_PLACEMENT_3D('',#77021,#38646,#38647);
#33367=AXIS2_PLACEMENT_3D('',#77026,#38649,#38650);
#33368=AXIS2_PLACEMENT_3D('',#77029,#38652,#38653);
#33369=AXIS2_PLACEMENT_3D('',#77030,#38654,#38655);
#33370=AXIS2_PLACEMENT_3D('',#77039,#38656,#38657);
#33371=AXIS2_PLACEMENT_3D('',#77040,#38658,#38659);
#33372=AXIS2_PLACEMENT_3D('',#77056,#38669,#38670);
#33373=AXIS2_PLACEMENT_3D('',#77057,#38671,#38672);
#33374=AXIS2_PLACEMENT_3D('',#77058,#38673,#38674);
#33375=AXIS2_PLACEMENT_3D('',#77060,#38675,#38676);
#33376=AXIS2_PLACEMENT_3D('',#77061,#38677,#38678);
#33377=AXIS2_PLACEMENT_3D('',#77062,#38679,#38680);
#33378=AXIS2_PLACEMENT_3D('',#77063,#38681,#38682);
#33379=AXIS2_PLACEMENT_3D('',#77065,#38683,#38684);
#33380=AXIS2_PLACEMENT_3D('',#77066,#38685,#38686);
#33381=AXIS2_PLACEMENT_3D('',#77070,#38688,#38689);
#33382=AXIS2_PLACEMENT_3D('',#77072,#38690,#38691);
#33383=AXIS2_PLACEMENT_3D('',#77073,#38692,#38693);
#33384=AXIS2_PLACEMENT_3D('',#77074,#38694,#38695);
#33385=AXIS2_PLACEMENT_3D('',#77078,#38697,#38698);
#33386=AXIS2_PLACEMENT_3D('',#77080,#38699,#38700);
#33387=AXIS2_PLACEMENT_3D('',#77081,#38701,#38702);
#33388=AXIS2_PLACEMENT_3D('',#77082,#38703,#38704);
#33389=AXIS2_PLACEMENT_3D('',#77090,#38710,#38711);
#33390=AXIS2_PLACEMENT_3D('',#77096,#38715,#38716);
#33391=AXIS2_PLACEMENT_3D('',#77099,#38717,#38718);
#33392=AXIS2_PLACEMENT_3D('',#77101,#38719,#38720);
#33393=AXIS2_PLACEMENT_3D('',#77103,#38722,#38723);
#33394=AXIS2_PLACEMENT_3D('',#77104,#38724,#38725);
#33395=AXIS2_PLACEMENT_3D('',#77108,#38728,#38729);
#33396=AXIS2_PLACEMENT_3D('',#77109,#38730,#38731);
#33397=AXIS2_PLACEMENT_3D('',#77110,#38732,#38733);
#33398=AXIS2_PLACEMENT_3D('',#77116,#38737,#38738);
#33399=AXIS2_PLACEMENT_3D('',#77119,#38739,#38740);
#33400=AXIS2_PLACEMENT_3D('',#77121,#38741,#38742);
#33401=AXIS2_PLACEMENT_3D('',#77123,#38744,#38745);
#33402=AXIS2_PLACEMENT_3D('',#77124,#38746,#38747);
#33403=AXIS2_PLACEMENT_3D('',#77128,#38750,#38751);
#33404=AXIS2_PLACEMENT_3D('',#77129,#38752,#38753);
#33405=AXIS2_PLACEMENT_3D('',#77130,#38754,#38755);
#33406=AXIS2_PLACEMENT_3D('',#77138,#38761,#38762);
#33407=AXIS2_PLACEMENT_3D('',#77142,#38765,#38766);
#33408=AXIS2_PLACEMENT_3D('',#77146,#38769,#38770);
#33409=AXIS2_PLACEMENT_3D('',#77148,#38772,#38773);
#33410=AXIS2_PLACEMENT_3D('',#77151,#38776,#38777);
#33411=AXIS2_PLACEMENT_3D('',#77152,#38778,#38779);
#38624=DIRECTION('axis',(0.,0.,1.));
#38625=DIRECTION('refdir',(1.,0.,0.));
#38626=DIRECTION('center_axis',(0.,-1.,0.));
#38627=DIRECTION('ref_axis',(-1.83697019872103E-16,0.,-1.));
#38628=DIRECTION('center_axis',(0.,-1.,0.));
#38629=DIRECTION('ref_axis',(1.,0.,0.));
#38630=DIRECTION('center_axis',(0.,1.,0.));
#38631=DIRECTION('ref_axis',(1.,0.,0.));
#38632=DIRECTION('center_axis',(0.,1.,0.));
#38633=DIRECTION('ref_axis',(1.,0.,0.));
#38634=DIRECTION('',(-1.,0.,0.));
#38635=DIRECTION('center_axis',(0.,-1.,0.));
#38636=DIRECTION('ref_axis',(1.,0.,0.));
#38637=DIRECTION('',(-1.,0.,0.));
#38638=DIRECTION('',(0.,0.,-1.));
#38639=DIRECTION('',(1.,0.,0.));
#38640=DIRECTION('',(0.,0.,1.));
#38641=DIRECTION('',(-1.,0.,0.));
#38642=DIRECTION('',(0.,0.,-1.));
#38643=DIRECTION('center_axis',(0.,1.,0.));
#38644=DIRECTION('ref_axis',(1.,0.,-4.93432455388958E-16));
#38645=DIRECTION('',(0.,0.,1.));
#38646=DIRECTION('center_axis',(0.,1.,0.));
#38647=DIRECTION('ref_axis',(-1.,0.,4.93432455388958E-16));
#38648=DIRECTION('',(0.,0.,-1.));
#38649=DIRECTION('center_axis',(0.,1.,0.));
#38650=DIRECTION('ref_axis',(1.,0.,-4.93432455388958E-16));
#38651=DIRECTION('',(0.,0.,1.));
#38652=DIRECTION('center_axis',(0.,1.,0.));
#38653=DIRECTION('ref_axis',(-1.,0.,4.93432455388958E-16));
#38654=DIRECTION('center_axis',(0.,-1.,0.));
#38655=DIRECTION('ref_axis',(-1.83697019872103E-16,0.,-1.));
#38656=DIRECTION('center_axis',(0.,1.,0.));
#38657=DIRECTION('ref_axis',(1.,0.,0.));
#38658=DIRECTION('center_axis',(0.,0.,1.));
#38659=DIRECTION('ref_axis',(1.,0.,0.));
#38660=DIRECTION('',(0.,1.,0.));
#38661=DIRECTION('',(1.,0.,0.));
#38662=DIRECTION('',(0.,1.,0.));
#38663=DIRECTION('',(0.,1.,0.));
#38664=DIRECTION('',(1.,0.,0.));
#38665=DIRECTION('',(0.,-1.,0.));
#38666=DIRECTION('',(0.,1.,0.));
#38667=DIRECTION('',(1.,0.,0.));
#38668=DIRECTION('',(0.,-1.,0.));
#38669=DIRECTION('center_axis',(0.,1.,0.));
#38670=DIRECTION('ref_axis',(5.0532154980743E-16,0.,-1.));
#38671=DIRECTION('center_axis',(0.,1.,0.));
#38672=DIRECTION('ref_axis',(1.,0.,0.));
#38673=DIRECTION('center_axis',(0.,1.,0.));
#38674=DIRECTION('ref_axis',(1.,0.,0.));
#38675=DIRECTION('center_axis',(0.,-1.,0.));
#38676=DIRECTION('ref_axis',(1.,0.,0.));
#38677=DIRECTION('center_axis',(0.,1.,0.));
#38678=DIRECTION('ref_axis',(-1.60812264967664E-16,0.,-1.));
#38679=DIRECTION('center_axis',(0.,1.,0.));
#38680=DIRECTION('ref_axis',(1.,0.,0.));
#38681=DIRECTION('center_axis',(0.,1.,0.));
#38682=DIRECTION('ref_axis',(1.,0.,0.));
#38683=DIRECTION('center_axis',(0.,-1.,0.));
#38684=DIRECTION('ref_axis',(1.,0.,0.));
#38685=DIRECTION('center_axis',(0.,1.,0.));
#38686=DIRECTION('ref_axis',(1.,0.,0.));
#38687=DIRECTION('',(0.,1.,0.));
#38688=DIRECTION('center_axis',(0.,-1.,0.));
#38689=DIRECTION('ref_axis',(1.,0.,0.));
#38690=DIRECTION('center_axis',(0.,-0.707106781186548,-0.707106781186548));
#38691=DIRECTION('ref_axis',(0.,0.707106781186548,-0.707106781186548));
#38692=DIRECTION('center_axis',(0.,-1.,0.));
#38693=DIRECTION('ref_axis',(1.,0.,0.));
#38694=DIRECTION('center_axis',(0.,1.,0.));
#38695=DIRECTION('ref_axis',(1.,0.,0.));
#38696=DIRECTION('',(0.,1.,0.));
#38697=DIRECTION('center_axis',(0.,-1.,0.));
#38698=DIRECTION('ref_axis',(1.,0.,0.));
#38699=DIRECTION('center_axis',(0.,-0.707106781186548,-0.707106781186548));
#38700=DIRECTION('ref_axis',(0.,0.707106781186548,-0.707106781186548));
#38701=DIRECTION('center_axis',(0.,-1.,0.));
#38702=DIRECTION('ref_axis',(1.,0.,0.));
#38703=DIRECTION('center_axis',(0.,0.707106781186548,0.707106781186548));
#38704=DIRECTION('ref_axis',(1.,0.,0.));
#38705=DIRECTION('',(-1.,0.,0.));
#38706=DIRECTION('',(-0.577350269189626,-0.577350269189626,0.577350269189626));
#38707=DIRECTION('',(0.577350269189624,-0.577350269189627,0.577350269189627));
#38708=DIRECTION('',(-1.,0.,0.));
#38709=DIRECTION('',(-1.,0.,0.));
#38710=DIRECTION('center_axis',(1.,0.,0.));
#38711=DIRECTION('ref_axis',(0.,0.,1.));
#38712=DIRECTION('',(0.,0.,1.));
#38713=DIRECTION('',(0.,-1.,0.));
#38714=DIRECTION('',(0.,-1.,0.));
#38715=DIRECTION('center_axis',(0.,-1.,0.));
#38716=DIRECTION('ref_axis',(1.,0.,-4.93432455388958E-16));
#38717=DIRECTION('center_axis',(0.,-0.707106781186548,0.707106781186548));
#38718=DIRECTION('ref_axis',(3.48909435263061E-16,0.707106781186547,0.707106781186547));
#38719=DIRECTION('center_axis',(0.,-1.,0.));
#38720=DIRECTION('ref_axis',(1.,0.,-4.93432455388958E-16));
#38721=DIRECTION('',(0.,-1.,0.));
#38722=DIRECTION('center_axis',(0.,-1.,0.));
#38723=DIRECTION('ref_axis',(1.,0.,-4.93432455388958E-16));
#38724=DIRECTION('center_axis',(-1.,0.,0.));
#38725=DIRECTION('ref_axis',(0.,0.,-1.));
#38726=DIRECTION('',(0.,0.,-1.));
#38727=DIRECTION('',(0.,-1.,0.));
#38728=DIRECTION('center_axis',(0.,-1.,0.));
#38729=DIRECTION('ref_axis',(-1.,0.,4.93432455388958E-16));
#38730=DIRECTION('center_axis',(0.,-1.,0.));
#38731=DIRECTION('ref_axis',(-1.,0.,4.93432455388958E-16));
#38732=DIRECTION('center_axis',(1.,0.,0.));
#38733=DIRECTION('ref_axis',(0.,0.,1.));
#38734=DIRECTION('',(0.,0.,1.));
#38735=DIRECTION('',(0.,-1.,0.));
#38736=DIRECTION('',(0.,-1.,0.));
#38737=DIRECTION('center_axis',(0.,-1.,0.));
#38738=DIRECTION('ref_axis',(1.,0.,-4.93432455388958E-16));
#38739=DIRECTION('center_axis',(0.,-0.707106781186548,0.707106781186548));
#38740=DIRECTION('ref_axis',(3.48909435263061E-16,0.707106781186547,0.707106781186547));
#38741=DIRECTION('center_axis',(0.,-1.,0.));
#38742=DIRECTION('ref_axis',(1.,0.,-4.93432455388958E-16));
#38743=DIRECTION('',(0.,-1.,0.));
#38744=DIRECTION('center_axis',(0.,-1.,0.));
#38745=DIRECTION('ref_axis',(1.,0.,-4.93432455388958E-16));
#38746=DIRECTION('center_axis',(-1.,0.,0.));
#38747=DIRECTION('ref_axis',(0.,0.,-1.));
#38748=DIRECTION('',(0.,0.,-1.));
#38749=DIRECTION('',(0.,-1.,0.));
#38750=DIRECTION('center_axis',(0.,-1.,0.));
#38751=DIRECTION('ref_axis',(-1.,0.,4.93432455388958E-16));
#38752=DIRECTION('center_axis',(0.,-1.,0.));
#38753=DIRECTION('ref_axis',(-1.,0.,4.93432455388958E-16));
#38754=DIRECTION('center_axis',(0.,1.,0.));
#38755=DIRECTION('ref_axis',(0.,0.,1.));
#38756=DIRECTION('',(0.,0.,1.));
#38757=DIRECTION('',(1.,0.,0.));
#38758=DIRECTION('',(1.,0.,0.));
#38759=DIRECTION('',(1.,0.,0.));
#38760=DIRECTION('',(0.,0.,-1.));
#38761=DIRECTION('center_axis',(0.707106781186548,0.707106781186548,0.));
#38762=DIRECTION('ref_axis',(0.,0.,-1.));
#38763=DIRECTION('',(0.,0.,-1.));
#38764=DIRECTION('',(0.577350269189626,-0.577350269189626,-0.577350269189626));
#38765=DIRECTION('center_axis',(-0.707106781186548,0.707106781186548,0.));
#38766=DIRECTION('ref_axis',(0.,0.,1.));
#38767=DIRECTION('',(-0.577350269189623,-0.577350269189626,-0.577350269189628));
#38768=DIRECTION('',(0.,0.,1.));
#38769=DIRECTION('center_axis',(0.,0.707106781186548,-0.707106781186548));
#38770=DIRECTION('ref_axis',(-1.,0.,0.));
#38771=DIRECTION('',(-1.,0.,0.));
#38772=DIRECTION('center_axis',(0.,0.,-1.));
#38773=DIRECTION('ref_axis',(-1.,0.,0.));
#38774=DIRECTION('',(0.,1.,0.));
#38775=DIRECTION('',(0.,1.,0.));
#38776=DIRECTION('center_axis',(1.,0.,0.));
#38777=DIRECTION('ref_axis',(0.,0.,-1.));
#38778=DIRECTION('center_axis',(-1.,0.,0.));
#38779=DIRECTION('ref_axis',(0.,0.,1.));
#76986=CARTESIAN_POINT('',(0.,0.,0.));
#76987=CARTESIAN_POINT('Origin',(10.,0.15,11.));
#76988=CARTESIAN_POINT('',(7.76393202250021,0.3,13.));
#76989=CARTESIAN_POINT('',(7.37511905031866,0.,13.));
#76990=CARTESIAN_POINT('Ctrl Pts',(7.76393202250021,0.3,13.));
#76991=CARTESIAN_POINT('Ctrl Pts',(7.57878298812804,0.16199805772513,13.));
#76992=CARTESIAN_POINT('Ctrl Pts',(7.37511905031866,3.46944695195361E-16,
13.));
#76993=CARTESIAN_POINT('',(12.6248809496813,0.,13.));
#76994=CARTESIAN_POINT('Origin',(10.,0.,11.));
#76995=CARTESIAN_POINT('',(12.2360679774998,0.3,13.));
#76996=CARTESIAN_POINT('Ctrl Pts',(12.6248809496813,3.46944695195361E-16,
13.));
#76997=CARTESIAN_POINT('Ctrl Pts',(12.421217011872,0.161998057725131,13.));
#76998=CARTESIAN_POINT('Ctrl Pts',(12.2360679774998,0.3,13.));
#76999=CARTESIAN_POINT('Origin',(10.,0.3,11.));
#77000=CARTESIAN_POINT('Origin',(0.,0.,0.800000000000001));
#77001=CARTESIAN_POINT('',(-7.37511905031866,0.,13.));
#77002=CARTESIAN_POINT('',(17.5,0.,13.));
#77003=CARTESIAN_POINT('',(-12.6248809496813,0.,13.));
#77004=CARTESIAN_POINT('Origin',(-10.,0.,11.));
#77005=CARTESIAN_POINT('',(-17.5,0.,13.));
#77006=CARTESIAN_POINT('',(17.5,0.,13.));
#77007=CARTESIAN_POINT('',(-17.5,0.,-11.4));
#77008=CARTESIAN_POINT('',(-17.5,0.,13.));
#77009=CARTESIAN_POINT('',(17.5,0.,-11.4));
#77010=CARTESIAN_POINT('',(-17.5,0.,-11.4));
#77011=CARTESIAN_POINT('',(17.5,0.,13.));
#77012=CARTESIAN_POINT('',(17.5,0.,-11.4));
#77013=CARTESIAN_POINT('',(17.5,0.,13.));
#77014=CARTESIAN_POINT('',(12.25,0.,-5.));
#77015=CARTESIAN_POINT('',(12.25,0.,-9.));
#77016=CARTESIAN_POINT('',(12.25,0.,-4.1));
#77017=CARTESIAN_POINT('',(7.75,0.,-9.));
#77018=CARTESIAN_POINT('Origin',(10.,0.,-9.));
#77019=CARTESIAN_POINT('',(7.75,0.,-5.));
#77020=CARTESIAN_POINT('',(7.75,0.,-2.1));
#77021=CARTESIAN_POINT('Origin',(10.,0.,-5.));
#77022=CARTESIAN_POINT('',(-7.75,0.,-5.));
#77023=CARTESIAN_POINT('',(-7.75,0.,-9.));
#77024=CARTESIAN_POINT('',(-7.75,0.,-4.1));
#77025=CARTESIAN_POINT('',(-12.25,0.,-9.));
#77026=CARTESIAN_POINT('Origin',(-10.,0.,-9.));
#77027=CARTESIAN_POINT('',(-12.25,0.,-5.));
#77028=CARTESIAN_POINT('',(-12.25,0.,-2.1));
#77029=CARTESIAN_POINT('Origin',(-10.,0.,-5.));
#77030=CARTESIAN_POINT('Origin',(-10.,0.15,11.));
#77031=CARTESIAN_POINT('',(-12.2360679774998,0.3,13.));
#77032=CARTESIAN_POINT('Ctrl Pts',(-12.2360679774998,0.3,13.));
#77033=CARTESIAN_POINT('Ctrl Pts',(-12.421217011872,0.161998057725133,13.));
#77034=CARTESIAN_POINT('Ctrl Pts',(-12.6248809496813,3.46944695195361E-16,
13.));
#77035=CARTESIAN_POINT('',(-7.76393202250021,0.3,13.));
#77036=CARTESIAN_POINT('Ctrl Pts',(-7.37511905031866,3.46944695195361E-16,
13.));
#77037=CARTESIAN_POINT('Ctrl Pts',(-7.57878298812804,0.161998057725129,
13.));
#77038=CARTESIAN_POINT('Ctrl Pts',(-7.76393202250021,0.3,13.));
#77039=CARTESIAN_POINT('Origin',(-10.,0.3,11.));
#77040=CARTESIAN_POINT('Origin',(-17.5,0.,13.));
#77041=CARTESIAN_POINT('',(17.5,9.5,13.));
#77042=CARTESIAN_POINT('',(17.5,0.,13.));
#77043=CARTESIAN_POINT('',(-17.5,9.5,13.));
#77044=CARTESIAN_POINT('',(-8.75,9.5,13.));
#77045=CARTESIAN_POINT('',(-17.5,0.,13.));
#77046=CARTESIAN_POINT('',(-12.2360679774998,3.5,13.));
#77047=CARTESIAN_POINT('',(-12.2360679774998,0.,13.));
#77048=CARTESIAN_POINT('',(-7.76393202250021,3.5,13.));
#77049=CARTESIAN_POINT('',(-13.75,3.5,13.));
#77050=CARTESIAN_POINT('',(-7.76393202250021,0.,13.));
#77051=CARTESIAN_POINT('',(7.76393202250021,3.5,13.));
#77052=CARTESIAN_POINT('',(7.76393202250021,0.,13.));
#77053=CARTESIAN_POINT('',(12.2360679774998,3.5,13.));
#77054=CARTESIAN_POINT('',(-3.75,3.5,13.));
#77055=CARTESIAN_POINT('',(12.2360679774998,0.,13.));
#77056=CARTESIAN_POINT('Origin',(-10.,0.,11.));
#77057=CARTESIAN_POINT('Origin',(-10.,3.5,11.));
#77058=CARTESIAN_POINT('Origin',(-10.,3.5,11.));
#77059=CARTESIAN_POINT('',(-11.7,3.5,11.));
#77060=CARTESIAN_POINT('Origin',(-10.,3.5,11.));
#77061=CARTESIAN_POINT('Origin',(10.,0.,11.));
#77062=CARTESIAN_POINT('Origin',(10.,3.5,11.));
#77063=CARTESIAN_POINT('Origin',(10.,3.5,11.));
#77064=CARTESIAN_POINT('',(8.3,3.5,11.));
#77065=CARTESIAN_POINT('Origin',(10.,3.5,11.));
#77066=CARTESIAN_POINT('Origin',(-10.,0.,11.));
#77067=CARTESIAN_POINT('',(-11.7,10.,11.));
#77068=CARTESIAN_POINT('',(-11.7,0.,11.));
#77069=CARTESIAN_POINT('',(-10.8,10.,12.5));
#77070=CARTESIAN_POINT('Origin',(-10.,10.,11.));
#77071=CARTESIAN_POINT('',(-9.2,10.,12.5));
#77072=CARTESIAN_POINT('Origin',(-10.,11.5,11.));
#77073=CARTESIAN_POINT('Origin',(-10.,10.,11.));
#77074=CARTESIAN_POINT('Origin',(10.,0.,11.));
#77075=CARTESIAN_POINT('',(8.3,10.,11.));
#77076=CARTESIAN_POINT('',(8.3,0.,11.));
#77077=CARTESIAN_POINT('',(9.2,10.,12.5));
#77078=CARTESIAN_POINT('Origin',(10.,10.,11.));
#77079=CARTESIAN_POINT('',(10.8,10.,12.5));
#77080=CARTESIAN_POINT('Origin',(10.,11.5,11.));
#77081=CARTESIAN_POINT('Origin',(10.,10.,11.));
#77082=CARTESIAN_POINT('Origin',(-8.75,9.75,12.75));
#77083=CARTESIAN_POINT('',(-17.,10.,12.5));
#77084=CARTESIAN_POINT('',(-8.75,10.,12.5));
#77085=CARTESIAN_POINT('',(-17.,10.,12.5));
#77086=CARTESIAN_POINT('',(17.,10.,12.5));
#77087=CARTESIAN_POINT('',(17.,10.,12.5));
#77088=CARTESIAN_POINT('',(-8.75,10.,12.5));
#77089=CARTESIAN_POINT('',(-8.75,10.,12.5));
#77090=CARTESIAN_POINT('Origin',(-7.75,10.,-9.));
#77091=CARTESIAN_POINT('',(-7.75,10.,-9.));
#77092=CARTESIAN_POINT('',(-7.75,10.,-5.));
#77093=CARTESIAN_POINT('',(-7.75,10.,-4.1));
#77094=CARTESIAN_POINT('',(-7.75,10.,-9.));
#77095=CARTESIAN_POINT('',(-7.75,10.,-5.));
#77096=CARTESIAN_POINT('Origin',(-10.,10.,-9.));
#77097=CARTESIAN_POINT('',(-11.2051970793194,10.,-10.9));
#77098=CARTESIAN_POINT('',(-8.79480292068061,10.,-10.9));
#77099=CARTESIAN_POINT('Origin',(-10.,11.9,-9.));
#77100=CARTESIAN_POINT('',(-12.25,10.,-9.));
#77101=CARTESIAN_POINT('Origin',(-10.,10.,-9.));
#77102=CARTESIAN_POINT('',(-12.25,10.,-9.));
#77103=CARTESIAN_POINT('Origin',(-10.,10.,-9.));
#77104=CARTESIAN_POINT('Origin',(-12.25,10.,-5.));
#77105=CARTESIAN_POINT('',(-12.25,10.,-5.));
#77106=CARTESIAN_POINT('',(-12.25,10.,-2.1));
#77107=CARTESIAN_POINT('',(-12.25,10.,-5.));
#77108=CARTESIAN_POINT('Origin',(-10.,10.,-5.));
#77109=CARTESIAN_POINT('Origin',(-10.,10.,-5.));
#77110=CARTESIAN_POINT('Origin',(12.25,10.,-9.));
#77111=CARTESIAN_POINT('',(12.25,10.,-9.));
#77112=CARTESIAN_POINT('',(12.25,10.,-5.));
#77113=CARTESIAN_POINT('',(12.25,10.,-4.1));
#77114=CARTESIAN_POINT('',(12.25,10.,-9.));
#77115=CARTESIAN_POINT('',(12.25,10.,-5.));
#77116=CARTESIAN_POINT('Origin',(10.,10.,-9.));
#77117=CARTESIAN_POINT('',(8.79480292068061,10.,-10.9));
#77118=CARTESIAN_POINT('',(11.2051970793194,10.,-10.9));
#77119=CARTESIAN_POINT('Origin',(10.,11.9,-9.));
#77120=CARTESIAN_POINT('',(7.75,10.,-9.));
#77121=CARTESIAN_POINT('Origin',(10.,10.,-9.));
#77122=CARTESIAN_POINT('',(7.75,10.,-9.));
#77123=CARTESIAN_POINT('Origin',(10.,10.,-9.));
#77124=CARTESIAN_POINT('Origin',(7.75,10.,-5.));
#77125=CARTESIAN_POINT('',(7.75,10.,-5.));
#77126=CARTESIAN_POINT('',(7.75,10.,-2.1));
#77127=CARTESIAN_POINT('',(7.75,10.,-5.));
#77128=CARTESIAN_POINT('Origin',(10.,10.,-5.));
#77129=CARTESIAN_POINT('Origin',(10.,10.,-5.));
#77130=CARTESIAN_POINT('Origin',(0.,10.,0.800000000000001));
#77131=CARTESIAN_POINT('',(17.,10.,-10.9));
#77132=CARTESIAN_POINT('',(17.,10.,6.9));
#77133=CARTESIAN_POINT('',(8.75,10.,-10.9));
#77134=CARTESIAN_POINT('',(8.75,10.,-10.9));
#77135=CARTESIAN_POINT('',(-17.,10.,-10.9));
#77136=CARTESIAN_POINT('',(8.75,10.,-10.9));
#77137=CARTESIAN_POINT('',(-17.,10.,-5.3));
#77138=CARTESIAN_POINT('Origin',(17.25,9.75,6.9));
#77139=CARTESIAN_POINT('',(17.5,9.5,-11.4));
#77140=CARTESIAN_POINT('',(17.5,9.5,6.9));
#77141=CARTESIAN_POINT('',(17.,10.,-10.9));
#77142=CARTESIAN_POINT('Origin',(-17.25,9.75,-5.3));
#77143=CARTESIAN_POINT('',(-17.5,9.5,-11.4));
#77144=CARTESIAN_POINT('',(-17.,10.,-10.9));
#77145=CARTESIAN_POINT('',(-17.5,9.5,-5.3));
#77146=CARTESIAN_POINT('Origin',(8.75,9.75,-11.15));
#77147=CARTESIAN_POINT('',(8.75,9.5,-11.4));
#77148=CARTESIAN_POINT('Origin',(17.5,0.,-11.4));
#77149=CARTESIAN_POINT('',(17.5,0.,-11.4));
#77150=CARTESIAN_POINT('',(-17.5,0.,-11.4));
#77151=CARTESIAN_POINT('Origin',(17.5,0.,13.));
#77152=CARTESIAN_POINT('Origin',(-17.5,0.,-11.4));
#135261=UNCERTAINTY_MEASURE_WITH_UNIT(LENGTH_MEASURE(0.01),#135283,
'DISTANCE_ACCURACY_VALUE',
'Maximum model space distance between geometric entities at asserted c
onnectivities');
#135267=UNCERTAINTY_MEASURE_WITH_UNIT(LENGTH_MEASURE(0.01),#135283,
'DISTANCE_ACCURACY_VALUE',
'Maximum model space distance between geometric entities at asserted c
onnectivities');
#135276=(
GEOMETRIC_REPRESENTATION_CONTEXT(3)
GLOBAL_UNCERTAINTY_ASSIGNED_CONTEXT((#135261))
GLOBAL_UNIT_ASSIGNED_CONTEXT((#135283,#135285,#135286))
REPRESENTATION_CONTEXT('','3D')
);
#135282=(
GEOMETRIC_REPRESENTATION_CONTEXT(3)
GLOBAL_UNCERTAINTY_ASSIGNED_CONTEXT((#135267))
GLOBAL_UNIT_ASSIGNED_CONTEXT((#135283,#135285,#135286))
REPRESENTATION_CONTEXT('','3D')
);
#135283=(
LENGTH_UNIT()
NAMED_UNIT(*)
SI_UNIT(.MILLI.,.METRE.)
);
#135285=(
NAMED_UNIT(*)
PLANE_ANGLE_UNIT()
SI_UNIT($,.RADIAN.)
);
#135286=(
NAMED_UNIT(*)
SI_UNIT($,.STERADIAN.)
SOLID_ANGLE_UNIT()
);
#135295=SHAPE_DEFINITION_REPRESENTATION(#135309,#135344);
#135309=PRODUCT_DEFINITION_SHAPE('',$,#135359);
#135344=SHAPE_REPRESENTATION('',(#33359),#135276);
#135350=PRODUCT_DEFINITION_CONTEXT('part definition',#135394,'design');
#135359=PRODUCT_DEFINITION('2026-10-15-19-09-11-263',
'Z-Axis L-Bracket Foot',#135373,#135350);
#135373=PRODUCT_DEFINITION_FORMATION('',$,#135404);
#135394=APPLICATION_CONTEXT(
'Core Data for Automotive Mechanical Design Process');
#135395=PRODUCT_CONTEXT('part definition',#135394,'mechanical');
#135404=PRODUCT('2026-10-15-19-09-11-263','Z-Axis L-Bracket Foot',$,(#135395));
#135418=PRESENTATION_STYLE_ASSIGNMENT((#135432));
#135432=SURFACE_STYLE_USAGE(.BOTH.,#135446);
#135446=SURFACE_SIDE_STYLE('',(#135460));
#135460=SURFACE_STYLE_FILL_AREA(#135474);
#135474=FILL_AREA_STYLE('Opaque(200,205,211)',(#135488));
#135488=FILL_AREA_STYLE_COLOUR('Opaque(200,205,211)',#135502);
#135502=COLOUR_RGB('Opaque(200,205,211)', 0.66274510, 0.83137255, 0.94901961);
ENDSEC;
END-ISO-10303-21;
